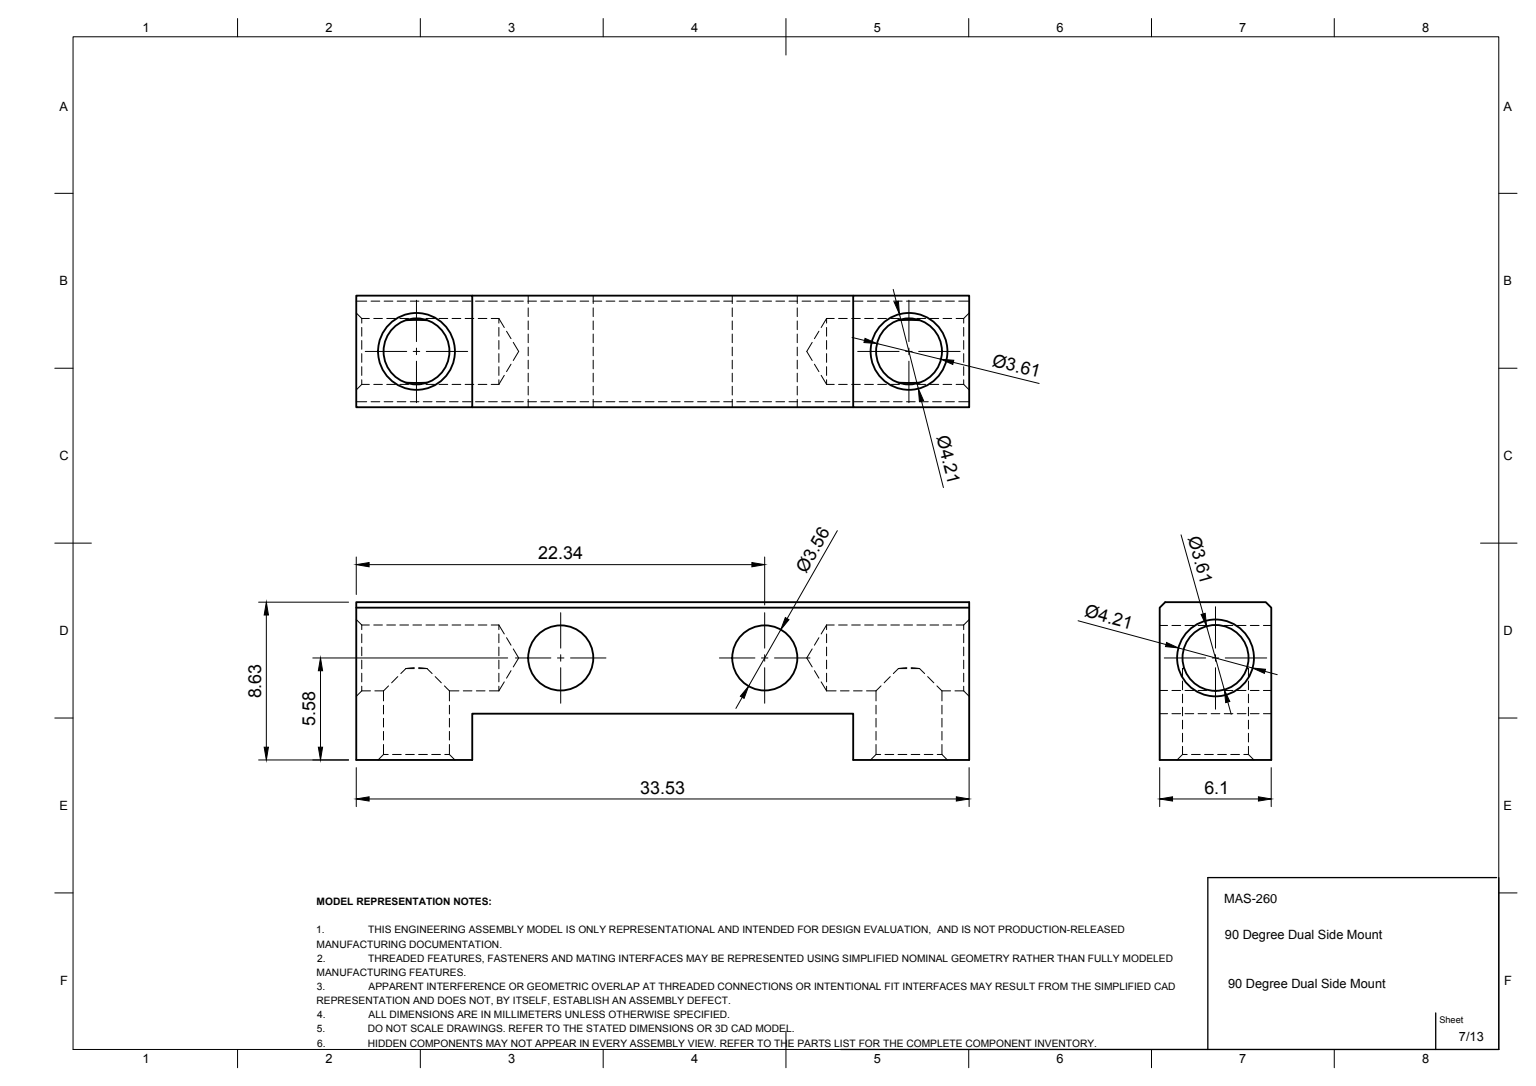
ISO-10303-21;
HEADER;
/* Generated by software containing ST-Developer
 * from STEP Tools, Inc. (www.steptools.com) 
 */

FILE_DESCRIPTION(
/* description */ (''),
/* implementation_level */ '2;1');

FILE_NAME(
/* name */ '90 Degree Dual Side Mount.step',
/* time_stamp */ '2026-10-15T13:29:10-07:00',
/* author */ (''),
/* organization */ (''),
/* preprocessor_version */ 'ST-DEVELOPER v20.2',
/* originating_system */ 'Autodesk Translation Framework v15.15.0.0',
/* authorisation */ '');

FILE_SCHEMA (('AUTOMOTIVE_DESIGN { 1 0 10303 214 3 1 1 }'));
ENDSEC;

DATA;
#10=MECHANICAL_DESIGN_GEOMETRIC_PRESENTATION_REPRESENTATION('',(#941),#83219);
#191=ELLIPSE('',#28417,2.5491199461775,1.8025);
#192=ELLIPSE('',#28419,2.5491199461775,1.8025);
#193=ELLIPSE('',#28421,2.5491199461775,1.8025);
#194=ELLIPSE('',#28427,2.5491199461775,1.8025);
#195=ELLIPSE('',#28429,2.5491199461775,1.8025);
#196=ELLIPSE('',#28431,2.5491199461775,1.8025);
#641=B_SPLINE_CURVE_WITH_KNOTS('',3,(#53054,#53055,#53056,#53057,#53058,
#53059,#53060),.UNSPECIFIED.,.F.,.F.,(4,3,4),(-0.0562125399722967,0.,0.0562125399722968),
 .UNSPECIFIED.);
#642=B_SPLINE_CURVE_WITH_KNOTS('',3,(#53062,#53063,#53064,#53065,#53066,
#53067),.UNSPECIFIED.,.F.,.F.,(4,2,4),(-0.961432950963571,-0.905220410991274,
-0.849007871018978),.UNSPECIFIED.);
#643=B_SPLINE_CURVE_WITH_KNOTS('',3,(#53077,#53078,#53079,#53080,#53081,
#53082,#53083),.UNSPECIFIED.,.F.,.F.,(4,3,4),(-0.0562125399722967,0.,0.0562125399722968),
 .UNSPECIFIED.);
#644=B_SPLINE_CURVE_WITH_KNOTS('',3,(#53085,#53086,#53087,#53088,#53089,
#53090),.UNSPECIFIED.,.F.,.F.,(4,2,4),(-0.961432950963571,-0.905220410991274,
-0.849007871018978),.UNSPECIFIED.);
#913=SHAPE_REPRESENTATION_RELATIONSHIP('SRR','None',#83308,#927);
#927=ADVANCED_BREP_SHAPE_REPRESENTATION('',(#955),#83213);
#941=STYLED_ITEM('',(#83387),#955);
#955=MANIFOLD_SOLID_BREP('Body1',#26937);
#1101=FACE_BOUND('',#4773,.T.);
#1102=FACE_BOUND('',#4777,.T.);
#1103=FACE_BOUND('',#4781,.T.);
#1104=FACE_BOUND('',#4785,.T.);
#1105=FACE_BOUND('',#4788,.T.);
#1106=FACE_BOUND('',#4792,.T.);
#1107=FACE_BOUND('',#4801,.T.);
#1108=FACE_BOUND('',#4802,.T.);
#1109=FACE_BOUND('',#4804,.T.);
#1110=FACE_BOUND('',#4805,.T.);
#1743=PLANE('',#28422);
#1744=PLANE('',#28432);
#1745=PLANE('',#28447);
#1746=PLANE('',#28451);
#1747=PLANE('',#28453);
#1748=PLANE('',#28454);
#1749=PLANE('',#28455);
#1750=PLANE('',#28456);
#1751=PLANE('',#28457);
#1752=PLANE('',#28458);
#1753=PLANE('',#28459);
#1754=PLANE('',#28460);
#2302=CYLINDRICAL_SURFACE('',#28407,1.778);
#2303=CYLINDRICAL_SURFACE('',#28410,1.778);
#2304=CYLINDRICAL_SURFACE('',#28416,1.8025);
#2305=CYLINDRICAL_SURFACE('',#28426,1.8025);
#2306=CYLINDRICAL_SURFACE('',#28435,1.8025);
#2307=CYLINDRICAL_SURFACE('',#28441,1.8025);
#3249=FACE_OUTER_BOUND('',#4768,.T.);
#3250=FACE_OUTER_BOUND('',#4769,.T.);
#3251=FACE_OUTER_BOUND('',#4770,.T.);
#3252=FACE_OUTER_BOUND('',#4771,.T.);
#3253=FACE_OUTER_BOUND('',#4772,.T.);
#3254=FACE_OUTER_BOUND('',#4774,.T.);
#3255=FACE_OUTER_BOUND('',#4775,.T.);
#3256=FACE_OUTER_BOUND('',#4776,.T.);
#3257=FACE_OUTER_BOUND('',#4778,.T.);
#3258=FACE_OUTER_BOUND('',#4779,.T.);
#3259=FACE_OUTER_BOUND('',#4780,.T.);
#3260=FACE_OUTER_BOUND('',#4782,.T.);
#3261=FACE_OUTER_BOUND('',#4783,.T.);
#3262=FACE_OUTER_BOUND('',#4784,.T.);
#3263=FACE_OUTER_BOUND('',#4786,.T.);
#3264=FACE_OUTER_BOUND('',#4787,.T.);
#3265=FACE_OUTER_BOUND('',#4789,.T.);
#3266=FACE_OUTER_BOUND('',#4790,.T.);
#3267=FACE_OUTER_BOUND('',#4791,.T.);
#3268=FACE_OUTER_BOUND('',#4793,.T.);
#3269=FACE_OUTER_BOUND('',#4794,.T.);
#3270=FACE_OUTER_BOUND('',#4795,.T.);
#3271=FACE_OUTER_BOUND('',#4796,.T.);
#3272=FACE_OUTER_BOUND('',#4797,.T.);
#3273=FACE_OUTER_BOUND('',#4798,.T.);
#3274=FACE_OUTER_BOUND('',#4799,.T.);
#3275=FACE_OUTER_BOUND('',#4800,.T.);
#3276=FACE_OUTER_BOUND('',#4803,.T.);
#4768=EDGE_LOOP('',(#22514,#22515,#22516,#22517));
#4769=EDGE_LOOP('',(#22518,#22519,#22520,#22521));
#4770=EDGE_LOOP('',(#22522,#22523,#22524,#22525));
#4771=EDGE_LOOP('',(#22526,#22527,#22528,#22529,#22530,#22531,#22532,#22533));
#4772=EDGE_LOOP('',(#22534,#22535,#22536,#22537));
#4773=EDGE_LOOP('',(#22538));
#4774=EDGE_LOOP('',(#22539,#22540,#22541,#22542));
#4775=EDGE_LOOP('',(#22543,#22544,#22545,#22546,#22547,#22548,#22549,#22550));
#4776=EDGE_LOOP('',(#22551,#22552,#22553,#22554));
#4777=EDGE_LOOP('',(#22555));
#4778=EDGE_LOOP('',(#22556,#22557));
#4779=EDGE_LOOP('',(#22558,#22559));
#4780=EDGE_LOOP('',(#22560,#22561,#22562,#22563,#22564));
#4781=EDGE_LOOP('',(#22565,#22566,#22567,#22568,#22569));
#4782=EDGE_LOOP('',(#22570,#22571));
#4783=EDGE_LOOP('',(#22572,#22573));
#4784=EDGE_LOOP('',(#22574,#22575,#22576,#22577,#22578));
#4785=EDGE_LOOP('',(#22579,#22580,#22581,#22582,#22583));
#4786=EDGE_LOOP('',(#22584,#22585,#22586,#22587));
#4787=EDGE_LOOP('',(#22588,#22589,#22590,#22591,#22592,#22593));
#4788=EDGE_LOOP('',(#22594));
#4789=EDGE_LOOP('',(#22595,#22596,#22597,#22598));
#4790=EDGE_LOOP('',(#22599,#22600,#22601,#22602));
#4791=EDGE_LOOP('',(#22603,#22604,#22605,#22606,#22607,#22608));
#4792=EDGE_LOOP('',(#22609));
#4793=EDGE_LOOP('',(#22610,#22611,#22612,#22613));
#4794=EDGE_LOOP('',(#22614,#22615,#22616,#22617));
#4795=EDGE_LOOP('',(#22618,#22619,#22620,#22621));
#4796=EDGE_LOOP('',(#22622,#22623,#22624,#22625));
#4797=EDGE_LOOP('',(#22626,#22627,#22628,#22629));
#4798=EDGE_LOOP('',(#22630,#22631,#22632,#22633));
#4799=EDGE_LOOP('',(#22634,#22635,#22636,#22637));
#4800=EDGE_LOOP('',(#22638,#22639,#22640,#22641,#22642,#22643,#22644,#22645));
#4801=EDGE_LOOP('',(#22646));
#4802=EDGE_LOOP('',(#22647));
#4803=EDGE_LOOP('',(#22648,#22649,#22650,#22651,#22652,#22653,#22654,#22655));
#4804=EDGE_LOOP('',(#22656));
#4805=EDGE_LOOP('',(#22657));
#7083=LINE('',#52991,#9594);
#7084=LINE('',#52997,#9595);
#7085=LINE('',#53003,#9596);
#7086=LINE('',#53007,#9597);
#7087=LINE('',#53020,#9598);
#7088=LINE('',#53022,#9599);
#7089=LINE('',#53024,#9600);
#7090=LINE('',#53025,#9601);
#7091=LINE('',#53030,#9602);
#7092=LINE('',#53034,#9603);
#7093=LINE('',#53047,#9604);
#7094=LINE('',#53049,#9605);
#7095=LINE('',#53051,#9606);
#7096=LINE('',#53052,#9607);
#7097=LINE('',#53072,#9608);
#7098=LINE('',#53095,#9609);
#7099=LINE('',#53101,#9610);
#7100=LINE('',#53106,#9611);
#7101=LINE('',#53108,#9612);
#7102=LINE('',#53110,#9613);
#7103=LINE('',#53111,#9614);
#7104=LINE('',#53112,#9615);
#7105=LINE('',#53115,#9616);
#7106=LINE('',#53118,#9617);
#7107=LINE('',#53123,#9618);
#7108=LINE('',#53124,#9619);
#7109=LINE('',#53126,#9620);
#7110=LINE('',#53128,#9621);
#7111=LINE('',#53129,#9622);
#7112=LINE('',#53132,#9623);
#7113=LINE('',#53134,#9624);
#7114=LINE('',#53135,#9625);
#7115=LINE('',#53137,#9626);
#7116=LINE('',#53139,#9627);
#7117=LINE('',#53142,#9628);
#7118=LINE('',#53144,#9629);
#7119=LINE('',#53145,#9630);
#7120=LINE('',#53148,#9631);
#7121=LINE('',#53150,#9632);
#7122=LINE('',#53151,#9633);
#7123=LINE('',#53153,#9634);
#7124=LINE('',#53154,#9635);
#9594=VECTOR('',#33683,1.778);
#9595=VECTOR('',#33690,1.778);
#9596=VECTOR('',#33697,1.9525);
#9597=VECTOR('',#33702,1.8025);
#9598=VECTOR('',#33715,10.);
#9599=VECTOR('',#33716,10.);
#9600=VECTOR('',#33717,10.);
#9601=VECTOR('',#33718,10.);
#9602=VECTOR('',#33723,1.9525);
#9603=VECTOR('',#33728,1.8025);
#9604=VECTOR('',#33741,10.);
#9605=VECTOR('',#33742,10.);
#9606=VECTOR('',#33743,10.);
#9607=VECTOR('',#33744,10.);
#9608=VECTOR('',#33753,1.8025);
#9609=VECTOR('',#33766,1.8025);
#9610=VECTOR('',#33773,1.9525);
#9611=VECTOR('',#33778,10.);
#9612=VECTOR('',#33779,10.);
#9613=VECTOR('',#33780,10.);
#9614=VECTOR('',#33781,10.);
#9615=VECTOR('',#33782,10.);
#9616=VECTOR('',#33785,1.8025);
#9617=VECTOR('',#33788,1.9525);
#9618=VECTOR('',#33793,10.);
#9619=VECTOR('',#33794,10.);
#9620=VECTOR('',#33795,10.);
#9621=VECTOR('',#33796,10.);
#9622=VECTOR('',#33797,10.);
#9623=VECTOR('',#33800,0.901250000000005);
#9624=VECTOR('',#33803,10.);
#9625=VECTOR('',#33804,10.);
#9626=VECTOR('',#33807,10.);
#9627=VECTOR('',#33810,10.);
#9628=VECTOR('',#33813,10.);
#9629=VECTOR('',#33814,10.);
#9630=VECTOR('',#33815,10.);
#9631=VECTOR('',#33818,10.);
#9632=VECTOR('',#33819,10.);
#9633=VECTOR('',#33820,10.);
#9634=VECTOR('',#33823,10.);
#9635=VECTOR('',#33824,10.);
#10740=CIRCLE('',#28408,1.778);
#10741=CIRCLE('',#28409,1.778);
#10742=CIRCLE('',#28411,1.778);
#10743=CIRCLE('',#28412,1.778);
#10744=CIRCLE('',#28414,1.8025);
#10745=CIRCLE('',#28415,2.1025);
#10746=CIRCLE('',#28418,1.8025);
#10747=CIRCLE('',#28420,1.8025);
#10748=CIRCLE('',#28424,1.8025);
#10749=CIRCLE('',#28425,2.1025);
#10750=CIRCLE('',#28428,1.8025);
#10751=CIRCLE('',#28430,1.8025);
#10752=CIRCLE('',#28436,1.8025);
#10753=CIRCLE('',#28437,1.8025);
#10754=CIRCLE('',#28438,1.8025);
#10755=CIRCLE('',#28442,1.8025);
#10756=CIRCLE('',#28443,1.8025);
#10757=CIRCLE('',#28444,1.8025);
#10758=CIRCLE('',#28446,2.1025);
#10759=CIRCLE('',#28450,2.1025);
#12651=VERTEX_POINT('',#52988);
#12652=VERTEX_POINT('',#52990);
#12653=VERTEX_POINT('',#52994);
#12654=VERTEX_POINT('',#52996);
#12655=VERTEX_POINT('',#53000);
#12656=VERTEX_POINT('',#53002);
#12657=VERTEX_POINT('',#53006);
#12658=VERTEX_POINT('',#53008);
#12659=VERTEX_POINT('',#53010);
#12660=VERTEX_POINT('',#53012);
#12661=VERTEX_POINT('',#53014);
#12662=VERTEX_POINT('',#53018);
#12663=VERTEX_POINT('',#53019);
#12664=VERTEX_POINT('',#53021);
#12665=VERTEX_POINT('',#53023);
#12666=VERTEX_POINT('',#53027);
#12667=VERTEX_POINT('',#53029);
#12668=VERTEX_POINT('',#53033);
#12669=VERTEX_POINT('',#53035);
#12670=VERTEX_POINT('',#53037);
#12671=VERTEX_POINT('',#53039);
#12672=VERTEX_POINT('',#53041);
#12673=VERTEX_POINT('',#53045);
#12674=VERTEX_POINT('',#53046);
#12675=VERTEX_POINT('',#53048);
#12676=VERTEX_POINT('',#53050);
#12677=VERTEX_POINT('',#53069);
#12678=VERTEX_POINT('',#53071);
#12679=VERTEX_POINT('',#53073);
#12680=VERTEX_POINT('',#53092);
#12681=VERTEX_POINT('',#53094);
#12682=VERTEX_POINT('',#53096);
#12683=VERTEX_POINT('',#53100);
#12684=VERTEX_POINT('',#53104);
#12685=VERTEX_POINT('',#53105);
#12686=VERTEX_POINT('',#53107);
#12687=VERTEX_POINT('',#53109);
#12688=VERTEX_POINT('',#53114);
#12689=VERTEX_POINT('',#53117);
#12690=VERTEX_POINT('',#53121);
#12691=VERTEX_POINT('',#53122);
#12692=VERTEX_POINT('',#53125);
#12693=VERTEX_POINT('',#53127);
#12694=VERTEX_POINT('',#53131);
#12695=VERTEX_POINT('',#53141);
#12696=VERTEX_POINT('',#53143);
#12697=VERTEX_POINT('',#53147);
#12698=VERTEX_POINT('',#53149);
#16118=EDGE_CURVE('',#12651,#12651,#10740,.T.);
#16119=EDGE_CURVE('',#12651,#12652,#7083,.T.);
#16120=EDGE_CURVE('',#12652,#12652,#10741,.T.);
#16121=EDGE_CURVE('',#12653,#12653,#10742,.T.);
#16122=EDGE_CURVE('',#12653,#12654,#7084,.T.);
#16123=EDGE_CURVE('',#12654,#12654,#10743,.T.);
#16124=EDGE_CURVE('',#12655,#12655,#10744,.T.);
#16125=EDGE_CURVE('',#12655,#12656,#7085,.T.);
#16126=EDGE_CURVE('',#12656,#12656,#10745,.T.);
#16127=EDGE_CURVE('',#12655,#12657,#7086,.T.);
#16128=EDGE_CURVE('',#12658,#12657,#191,.T.);
#16129=EDGE_CURVE('',#12658,#12659,#10746,.T.);
#16130=EDGE_CURVE('',#12660,#12659,#192,.T.);
#16131=EDGE_CURVE('',#12660,#12661,#10747,.T.);
#16132=EDGE_CURVE('',#12657,#12661,#193,.T.);
#16133=EDGE_CURVE('',#12662,#12663,#7087,.T.);
#16134=EDGE_CURVE('',#12663,#12664,#7088,.T.);
#16135=EDGE_CURVE('',#12665,#12664,#7089,.T.);
#16136=EDGE_CURVE('',#12662,#12665,#7090,.T.);
#16137=EDGE_CURVE('',#12666,#12666,#10748,.T.);
#16138=EDGE_CURVE('',#12666,#12667,#7091,.T.);
#16139=EDGE_CURVE('',#12667,#12667,#10749,.T.);
#16140=EDGE_CURVE('',#12666,#12668,#7092,.T.);
#16141=EDGE_CURVE('',#12669,#12668,#194,.T.);
#16142=EDGE_CURVE('',#12669,#12670,#10750,.T.);
#16143=EDGE_CURVE('',#12671,#12670,#195,.T.);
#16144=EDGE_CURVE('',#12671,#12672,#10751,.T.);
#16145=EDGE_CURVE('',#12668,#12672,#196,.T.);
#16146=EDGE_CURVE('',#12673,#12674,#7093,.T.);
#16147=EDGE_CURVE('',#12674,#12675,#7094,.T.);
#16148=EDGE_CURVE('',#12676,#12675,#7095,.T.);
#16149=EDGE_CURVE('',#12673,#12676,#7096,.T.);
#16150=EDGE_CURVE('',#12659,#12658,#641,.T.);
#16151=EDGE_CURVE('',#12661,#12660,#642,.T.);
#16152=EDGE_CURVE('',#12677,#12677,#10752,.T.);
#16153=EDGE_CURVE('',#12677,#12678,#7097,.T.);
#16154=EDGE_CURVE('',#12678,#12679,#10753,.T.);
#16155=EDGE_CURVE('',#12679,#12678,#10754,.T.);
#16156=EDGE_CURVE('',#12672,#12671,#643,.T.);
#16157=EDGE_CURVE('',#12670,#12669,#644,.T.);
#16158=EDGE_CURVE('',#12680,#12680,#10755,.T.);
#16159=EDGE_CURVE('',#12680,#12681,#7098,.T.);
#16160=EDGE_CURVE('',#12681,#12682,#10756,.T.);
#16161=EDGE_CURVE('',#12682,#12681,#10757,.T.);
#16162=EDGE_CURVE('',#12677,#12683,#7099,.T.);
#16163=EDGE_CURVE('',#12683,#12683,#10758,.T.);
#16164=EDGE_CURVE('',#12684,#12685,#7100,.T.);
#16165=EDGE_CURVE('',#12686,#12684,#7101,.T.);
#16166=EDGE_CURVE('',#12687,#12686,#7102,.T.);
#16167=EDGE_CURVE('',#12687,#12662,#7103,.T.);
#16168=EDGE_CURVE('',#12685,#12665,#7104,.T.);
#16169=EDGE_CURVE('',#12688,#12679,#7105,.T.);
#16170=EDGE_CURVE('',#12680,#12689,#7106,.T.);
#16171=EDGE_CURVE('',#12689,#12689,#10759,.T.);
#16172=EDGE_CURVE('',#12690,#12691,#7107,.T.);
#16173=EDGE_CURVE('',#12675,#12690,#7108,.T.);
#16174=EDGE_CURVE('',#12674,#12692,#7109,.T.);
#16175=EDGE_CURVE('',#12693,#12692,#7110,.T.);
#16176=EDGE_CURVE('',#12693,#12691,#7111,.T.);
#16177=EDGE_CURVE('',#12694,#12682,#7112,.T.);
#16178=EDGE_CURVE('',#12685,#12690,#7113,.T.);
#16179=EDGE_CURVE('',#12691,#12684,#7114,.T.);
#16180=EDGE_CURVE('',#12686,#12693,#7115,.T.);
#16181=EDGE_CURVE('',#12692,#12687,#7116,.T.);
#16182=EDGE_CURVE('',#12695,#12673,#7117,.T.);
#16183=EDGE_CURVE('',#12696,#12676,#7118,.T.);
#16184=EDGE_CURVE('',#12695,#12696,#7119,.T.);
#16185=EDGE_CURVE('',#12697,#12695,#7120,.T.);
#16186=EDGE_CURVE('',#12698,#12696,#7121,.T.);
#16187=EDGE_CURVE('',#12697,#12698,#7122,.T.);
#16188=EDGE_CURVE('',#12663,#12697,#7123,.T.);
#16189=EDGE_CURVE('',#12664,#12698,#7124,.T.);
#22514=ORIENTED_EDGE('',*,*,#16118,.F.);
#22515=ORIENTED_EDGE('',*,*,#16119,.T.);
#22516=ORIENTED_EDGE('',*,*,#16120,.F.);
#22517=ORIENTED_EDGE('',*,*,#16119,.F.);
#22518=ORIENTED_EDGE('',*,*,#16121,.F.);
#22519=ORIENTED_EDGE('',*,*,#16122,.T.);
#22520=ORIENTED_EDGE('',*,*,#16123,.F.);
#22521=ORIENTED_EDGE('',*,*,#16122,.F.);
#22522=ORIENTED_EDGE('',*,*,#16124,.T.);
#22523=ORIENTED_EDGE('',*,*,#16125,.T.);
#22524=ORIENTED_EDGE('',*,*,#16126,.T.);
#22525=ORIENTED_EDGE('',*,*,#16125,.F.);
#22526=ORIENTED_EDGE('',*,*,#16124,.F.);
#22527=ORIENTED_EDGE('',*,*,#16127,.T.);
#22528=ORIENTED_EDGE('',*,*,#16128,.F.);
#22529=ORIENTED_EDGE('',*,*,#16129,.T.);
#22530=ORIENTED_EDGE('',*,*,#16130,.F.);
#22531=ORIENTED_EDGE('',*,*,#16131,.T.);
#22532=ORIENTED_EDGE('',*,*,#16132,.F.);
#22533=ORIENTED_EDGE('',*,*,#16127,.F.);
#22534=ORIENTED_EDGE('',*,*,#16133,.T.);
#22535=ORIENTED_EDGE('',*,*,#16134,.T.);
#22536=ORIENTED_EDGE('',*,*,#16135,.F.);
#22537=ORIENTED_EDGE('',*,*,#16136,.F.);
#22538=ORIENTED_EDGE('',*,*,#16126,.F.);
#22539=ORIENTED_EDGE('',*,*,#16137,.T.);
#22540=ORIENTED_EDGE('',*,*,#16138,.T.);
#22541=ORIENTED_EDGE('',*,*,#16139,.T.);
#22542=ORIENTED_EDGE('',*,*,#16138,.F.);
#22543=ORIENTED_EDGE('',*,*,#16137,.F.);
#22544=ORIENTED_EDGE('',*,*,#16140,.T.);
#22545=ORIENTED_EDGE('',*,*,#16141,.F.);
#22546=ORIENTED_EDGE('',*,*,#16142,.T.);
#22547=ORIENTED_EDGE('',*,*,#16143,.F.);
#22548=ORIENTED_EDGE('',*,*,#16144,.T.);
#22549=ORIENTED_EDGE('',*,*,#16145,.F.);
#22550=ORIENTED_EDGE('',*,*,#16140,.F.);
#22551=ORIENTED_EDGE('',*,*,#16146,.T.);
#22552=ORIENTED_EDGE('',*,*,#16147,.T.);
#22553=ORIENTED_EDGE('',*,*,#16148,.F.);
#22554=ORIENTED_EDGE('',*,*,#16149,.F.);
#22555=ORIENTED_EDGE('',*,*,#16139,.F.);
#22556=ORIENTED_EDGE('',*,*,#16150,.F.);
#22557=ORIENTED_EDGE('',*,*,#16129,.F.);
#22558=ORIENTED_EDGE('',*,*,#16151,.F.);
#22559=ORIENTED_EDGE('',*,*,#16131,.F.);
#22560=ORIENTED_EDGE('',*,*,#16152,.F.);
#22561=ORIENTED_EDGE('',*,*,#16153,.T.);
#22562=ORIENTED_EDGE('',*,*,#16154,.T.);
#22563=ORIENTED_EDGE('',*,*,#16155,.T.);
#22564=ORIENTED_EDGE('',*,*,#16153,.F.);
#22565=ORIENTED_EDGE('',*,*,#16151,.T.);
#22566=ORIENTED_EDGE('',*,*,#16130,.T.);
#22567=ORIENTED_EDGE('',*,*,#16150,.T.);
#22568=ORIENTED_EDGE('',*,*,#16128,.T.);
#22569=ORIENTED_EDGE('',*,*,#16132,.T.);
#22570=ORIENTED_EDGE('',*,*,#16156,.F.);
#22571=ORIENTED_EDGE('',*,*,#16144,.F.);
#22572=ORIENTED_EDGE('',*,*,#16157,.F.);
#22573=ORIENTED_EDGE('',*,*,#16142,.F.);
#22574=ORIENTED_EDGE('',*,*,#16158,.F.);
#22575=ORIENTED_EDGE('',*,*,#16159,.T.);
#22576=ORIENTED_EDGE('',*,*,#16160,.T.);
#22577=ORIENTED_EDGE('',*,*,#16161,.T.);
#22578=ORIENTED_EDGE('',*,*,#16159,.F.);
#22579=ORIENTED_EDGE('',*,*,#16157,.T.);
#22580=ORIENTED_EDGE('',*,*,#16141,.T.);
#22581=ORIENTED_EDGE('',*,*,#16145,.T.);
#22582=ORIENTED_EDGE('',*,*,#16156,.T.);
#22583=ORIENTED_EDGE('',*,*,#16143,.T.);
#22584=ORIENTED_EDGE('',*,*,#16152,.T.);
#22585=ORIENTED_EDGE('',*,*,#16162,.T.);
#22586=ORIENTED_EDGE('',*,*,#16163,.T.);
#22587=ORIENTED_EDGE('',*,*,#16162,.F.);
#22588=ORIENTED_EDGE('',*,*,#16164,.F.);
#22589=ORIENTED_EDGE('',*,*,#16165,.F.);
#22590=ORIENTED_EDGE('',*,*,#16166,.F.);
#22591=ORIENTED_EDGE('',*,*,#16167,.T.);
#22592=ORIENTED_EDGE('',*,*,#16136,.T.);
#22593=ORIENTED_EDGE('',*,*,#16168,.F.);
#22594=ORIENTED_EDGE('',*,*,#16163,.F.);
#22595=ORIENTED_EDGE('',*,*,#16169,.T.);
#22596=ORIENTED_EDGE('',*,*,#16154,.F.);
#22597=ORIENTED_EDGE('',*,*,#16155,.F.);
#22598=ORIENTED_EDGE('',*,*,#16169,.F.);
#22599=ORIENTED_EDGE('',*,*,#16158,.T.);
#22600=ORIENTED_EDGE('',*,*,#16170,.T.);
#22601=ORIENTED_EDGE('',*,*,#16171,.T.);
#22602=ORIENTED_EDGE('',*,*,#16170,.F.);
#22603=ORIENTED_EDGE('',*,*,#16172,.F.);
#22604=ORIENTED_EDGE('',*,*,#16173,.F.);
#22605=ORIENTED_EDGE('',*,*,#16147,.F.);
#22606=ORIENTED_EDGE('',*,*,#16174,.T.);
#22607=ORIENTED_EDGE('',*,*,#16175,.F.);
#22608=ORIENTED_EDGE('',*,*,#16176,.T.);
#22609=ORIENTED_EDGE('',*,*,#16171,.F.);
#22610=ORIENTED_EDGE('',*,*,#16177,.T.);
#22611=ORIENTED_EDGE('',*,*,#16160,.F.);
#22612=ORIENTED_EDGE('',*,*,#16161,.F.);
#22613=ORIENTED_EDGE('',*,*,#16177,.F.);
#22614=ORIENTED_EDGE('',*,*,#16164,.T.);
#22615=ORIENTED_EDGE('',*,*,#16178,.T.);
#22616=ORIENTED_EDGE('',*,*,#16172,.T.);
#22617=ORIENTED_EDGE('',*,*,#16179,.T.);
#22618=ORIENTED_EDGE('',*,*,#16179,.F.);
#22619=ORIENTED_EDGE('',*,*,#16176,.F.);
#22620=ORIENTED_EDGE('',*,*,#16180,.F.);
#22621=ORIENTED_EDGE('',*,*,#16165,.T.);
#22622=ORIENTED_EDGE('',*,*,#16166,.T.);
#22623=ORIENTED_EDGE('',*,*,#16180,.T.);
#22624=ORIENTED_EDGE('',*,*,#16175,.T.);
#22625=ORIENTED_EDGE('',*,*,#16181,.T.);
#22626=ORIENTED_EDGE('',*,*,#16182,.T.);
#22627=ORIENTED_EDGE('',*,*,#16149,.T.);
#22628=ORIENTED_EDGE('',*,*,#16183,.F.);
#22629=ORIENTED_EDGE('',*,*,#16184,.F.);
#22630=ORIENTED_EDGE('',*,*,#16185,.T.);
#22631=ORIENTED_EDGE('',*,*,#16184,.T.);
#22632=ORIENTED_EDGE('',*,*,#16186,.F.);
#22633=ORIENTED_EDGE('',*,*,#16187,.F.);
#22634=ORIENTED_EDGE('',*,*,#16188,.T.);
#22635=ORIENTED_EDGE('',*,*,#16187,.T.);
#22636=ORIENTED_EDGE('',*,*,#16189,.F.);
#22637=ORIENTED_EDGE('',*,*,#16134,.F.);
#22638=ORIENTED_EDGE('',*,*,#16178,.F.);
#22639=ORIENTED_EDGE('',*,*,#16168,.T.);
#22640=ORIENTED_EDGE('',*,*,#16135,.T.);
#22641=ORIENTED_EDGE('',*,*,#16189,.T.);
#22642=ORIENTED_EDGE('',*,*,#16186,.T.);
#22643=ORIENTED_EDGE('',*,*,#16183,.T.);
#22644=ORIENTED_EDGE('',*,*,#16148,.T.);
#22645=ORIENTED_EDGE('',*,*,#16173,.T.);
#22646=ORIENTED_EDGE('',*,*,#16120,.T.);
#22647=ORIENTED_EDGE('',*,*,#16123,.T.);
#22648=ORIENTED_EDGE('',*,*,#16181,.F.);
#22649=ORIENTED_EDGE('',*,*,#16174,.F.);
#22650=ORIENTED_EDGE('',*,*,#16146,.F.);
#22651=ORIENTED_EDGE('',*,*,#16182,.F.);
#22652=ORIENTED_EDGE('',*,*,#16185,.F.);
#22653=ORIENTED_EDGE('',*,*,#16188,.F.);
#22654=ORIENTED_EDGE('',*,*,#16133,.F.);
#22655=ORIENTED_EDGE('',*,*,#16167,.F.);
#22656=ORIENTED_EDGE('',*,*,#16118,.T.);
#22657=ORIENTED_EDGE('',*,*,#16121,.T.);
#25526=CONICAL_SURFACE('',#28413,1.9525,0.785398163397452);
#25527=CONICAL_SURFACE('',#28423,1.9525,0.785398163397452);
#25528=CONICAL_SURFACE('',#28433,0.90125,1.02974425867665);
#25529=CONICAL_SURFACE('',#28434,0.90125,1.02974425867665);
#25530=CONICAL_SURFACE('',#28439,0.90125,1.02974425867665);
#25531=CONICAL_SURFACE('',#28440,0.90125,1.02974425867665);
#25532=CONICAL_SURFACE('',#28445,1.9525,0.785398163397448);
#25533=CONICAL_SURFACE('',#28448,1.8025,1.02974425867665);
#25534=CONICAL_SURFACE('',#28449,1.9525,0.785398163397448);
#25535=CONICAL_SURFACE('',#28452,0.901250000000005,1.02974425867665);
#26442=ADVANCED_FACE('',(#3249),#2302,.F.);
#26443=ADVANCED_FACE('',(#3250),#2303,.F.);
#26444=ADVANCED_FACE('',(#3251),#25526,.F.);
#26445=ADVANCED_FACE('',(#3252),#2304,.F.);
#26446=ADVANCED_FACE('',(#3253,#1101),#1743,.T.);
#26447=ADVANCED_FACE('',(#3254),#25527,.F.);
#26448=ADVANCED_FACE('',(#3255),#2305,.F.);
#26449=ADVANCED_FACE('',(#3256,#1102),#1744,.T.);
#26450=ADVANCED_FACE('',(#3257),#25528,.F.);
#26451=ADVANCED_FACE('',(#3258),#25529,.F.);
#26452=ADVANCED_FACE('',(#3259,#1103),#2306,.F.);
#26453=ADVANCED_FACE('',(#3260),#25530,.F.);
#26454=ADVANCED_FACE('',(#3261),#25531,.F.);
#26455=ADVANCED_FACE('',(#3262,#1104),#2307,.F.);
#26456=ADVANCED_FACE('',(#3263),#25532,.F.);
#26457=ADVANCED_FACE('',(#3264,#1105),#1745,.T.);
#26458=ADVANCED_FACE('',(#3265),#25533,.F.);
#26459=ADVANCED_FACE('',(#3266),#25534,.F.);
#26460=ADVANCED_FACE('',(#3267,#1106),#1746,.T.);
#26461=ADVANCED_FACE('',(#3268),#25535,.F.);
#26462=ADVANCED_FACE('',(#3269),#1747,.T.);
#26463=ADVANCED_FACE('',(#3270),#1748,.T.);
#26464=ADVANCED_FACE('',(#3271),#1749,.T.);
#26465=ADVANCED_FACE('',(#3272),#1750,.T.);
#26466=ADVANCED_FACE('',(#3273),#1751,.T.);
#26467=ADVANCED_FACE('',(#3274),#1752,.T.);
#26468=ADVANCED_FACE('',(#3275,#1107,#1108),#1753,.T.);
#26469=ADVANCED_FACE('',(#3276,#1109,#1110),#1754,.F.);
#26937=CLOSED_SHELL('',(#26442,#26443,#26444,#26445,#26446,#26447,#26448,
#26449,#26450,#26451,#26452,#26453,#26454,#26455,#26456,#26457,#26458,#26459,
#26460,#26461,#26462,#26463,#26464,#26465,#26466,#26467,#26468,#26469));
#28406=AXIS2_PLACEMENT_3D('',#52986,#33677,#33678);
#28407=AXIS2_PLACEMENT_3D('',#52987,#33679,#33680);
#28408=AXIS2_PLACEMENT_3D('',#52989,#33681,#33682);
#28409=AXIS2_PLACEMENT_3D('',#52992,#33684,#33685);
#28410=AXIS2_PLACEMENT_3D('',#52993,#33686,#33687);
#28411=AXIS2_PLACEMENT_3D('',#52995,#33688,#33689);
#28412=AXIS2_PLACEMENT_3D('',#52998,#33691,#33692);
#28413=AXIS2_PLACEMENT_3D('',#52999,#33693,#33694);
#28414=AXIS2_PLACEMENT_3D('',#53001,#33695,#33696);
#28415=AXIS2_PLACEMENT_3D('',#53004,#33698,#33699);
#28416=AXIS2_PLACEMENT_3D('',#53005,#33700,#33701);
#28417=AXIS2_PLACEMENT_3D('',#53009,#33703,#33704);
#28418=AXIS2_PLACEMENT_3D('',#53011,#33705,#33706);
#28419=AXIS2_PLACEMENT_3D('',#53013,#33707,#33708);
#28420=AXIS2_PLACEMENT_3D('',#53015,#33709,#33710);
#28421=AXIS2_PLACEMENT_3D('',#53016,#33711,#33712);
#28422=AXIS2_PLACEMENT_3D('',#53017,#33713,#33714);
#28423=AXIS2_PLACEMENT_3D('',#53026,#33719,#33720);
#28424=AXIS2_PLACEMENT_3D('',#53028,#33721,#33722);
#28425=AXIS2_PLACEMENT_3D('',#53031,#33724,#33725);
#28426=AXIS2_PLACEMENT_3D('',#53032,#33726,#33727);
#28427=AXIS2_PLACEMENT_3D('',#53036,#33729,#33730);
#28428=AXIS2_PLACEMENT_3D('',#53038,#33731,#33732);
#28429=AXIS2_PLACEMENT_3D('',#53040,#33733,#33734);
#28430=AXIS2_PLACEMENT_3D('',#53042,#33735,#33736);
#28431=AXIS2_PLACEMENT_3D('',#53043,#33737,#33738);
#28432=AXIS2_PLACEMENT_3D('',#53044,#33739,#33740);
#28433=AXIS2_PLACEMENT_3D('',#53053,#33745,#33746);
#28434=AXIS2_PLACEMENT_3D('',#53061,#33747,#33748);
#28435=AXIS2_PLACEMENT_3D('',#53068,#33749,#33750);
#28436=AXIS2_PLACEMENT_3D('',#53070,#33751,#33752);
#28437=AXIS2_PLACEMENT_3D('',#53074,#33754,#33755);
#28438=AXIS2_PLACEMENT_3D('',#53075,#33756,#33757);
#28439=AXIS2_PLACEMENT_3D('',#53076,#33758,#33759);
#28440=AXIS2_PLACEMENT_3D('',#53084,#33760,#33761);
#28441=AXIS2_PLACEMENT_3D('',#53091,#33762,#33763);
#28442=AXIS2_PLACEMENT_3D('',#53093,#33764,#33765);
#28443=AXIS2_PLACEMENT_3D('',#53097,#33767,#33768);
#28444=AXIS2_PLACEMENT_3D('',#53098,#33769,#33770);
#28445=AXIS2_PLACEMENT_3D('',#53099,#33771,#33772);
#28446=AXIS2_PLACEMENT_3D('',#53102,#33774,#33775);
#28447=AXIS2_PLACEMENT_3D('',#53103,#33776,#33777);
#28448=AXIS2_PLACEMENT_3D('',#53113,#33783,#33784);
#28449=AXIS2_PLACEMENT_3D('',#53116,#33786,#33787);
#28450=AXIS2_PLACEMENT_3D('',#53119,#33789,#33790);
#28451=AXIS2_PLACEMENT_3D('',#53120,#33791,#33792);
#28452=AXIS2_PLACEMENT_3D('',#53130,#33798,#33799);
#28453=AXIS2_PLACEMENT_3D('',#53133,#33801,#33802);
#28454=AXIS2_PLACEMENT_3D('',#53136,#33805,#33806);
#28455=AXIS2_PLACEMENT_3D('',#53138,#33808,#33809);
#28456=AXIS2_PLACEMENT_3D('',#53140,#33811,#33812);
#28457=AXIS2_PLACEMENT_3D('',#53146,#33816,#33817);
#28458=AXIS2_PLACEMENT_3D('',#53152,#33821,#33822);
#28459=AXIS2_PLACEMENT_3D('',#53155,#33825,#33826);
#28460=AXIS2_PLACEMENT_3D('',#53156,#33827,#33828);
#33677=DIRECTION('axis',(0.,0.,1.));
#33678=DIRECTION('refdir',(1.,0.,0.));
#33679=DIRECTION('center_axis',(0.,0.,1.));
#33680=DIRECTION('ref_axis',(1.,0.,0.));
#33681=DIRECTION('center_axis',(0.,0.,1.));
#33682=DIRECTION('ref_axis',(1.,0.,0.));
#33683=DIRECTION('',(0.,0.,1.));
#33684=DIRECTION('center_axis',(0.,0.,-1.));
#33685=DIRECTION('ref_axis',(1.,0.,0.));
#33686=DIRECTION('center_axis',(0.,0.,1.));
#33687=DIRECTION('ref_axis',(1.,0.,0.));
#33688=DIRECTION('center_axis',(0.,0.,1.));
#33689=DIRECTION('ref_axis',(1.,0.,0.));
#33690=DIRECTION('',(0.,0.,1.));
#33691=DIRECTION('center_axis',(0.,0.,-1.));
#33692=DIRECTION('ref_axis',(1.,0.,0.));
#33693=DIRECTION('center_axis',(0.,-1.,0.));
#33694=DIRECTION('ref_axis',(1.,0.,0.));
#33695=DIRECTION('center_axis',(0.,1.,0.));
#33696=DIRECTION('ref_axis',(1.,0.,0.));
#33697=DIRECTION('',(-0.70710678118655,-0.707106781186545,-8.65956056235497E-17));
#33698=DIRECTION('center_axis',(0.,-1.,0.));
#33699=DIRECTION('ref_axis',(1.,0.,0.));
#33700=DIRECTION('center_axis',(0.,1.,0.));
#33701=DIRECTION('ref_axis',(1.,0.,0.));
#33702=DIRECTION('',(0.,1.,0.));
#33703=DIRECTION('center_axis',(0.707106781186548,-0.707106781186548,0.));
#33704=DIRECTION('ref_axis',(0.707106781186548,0.707106781186548,0.));
#33705=DIRECTION('center_axis',(0.,1.,0.));
#33706=DIRECTION('ref_axis',(1.,0.,0.));
#33707=DIRECTION('center_axis',(-0.707106781186548,-0.707106781186548,0.));
#33708=DIRECTION('ref_axis',(0.707106781186548,-0.707106781186548,0.));
#33709=DIRECTION('center_axis',(0.,1.,0.));
#33710=DIRECTION('ref_axis',(1.,0.,0.));
#33711=DIRECTION('center_axis',(0.707106781186548,-0.707106781186548,0.));
#33712=DIRECTION('ref_axis',(0.707106781186548,0.707106781186548,0.));
#33713=DIRECTION('center_axis',(0.,-1.,0.));
#33714=DIRECTION('ref_axis',(1.,0.,0.));
#33715=DIRECTION('',(1.,0.,0.));
#33716=DIRECTION('',(0.,0.,1.));
#33717=DIRECTION('',(1.,0.,0.));
#33718=DIRECTION('',(0.,0.,1.));
#33719=DIRECTION('center_axis',(0.,-1.,0.));
#33720=DIRECTION('ref_axis',(1.,0.,0.));
#33721=DIRECTION('center_axis',(0.,1.,0.));
#33722=DIRECTION('ref_axis',(1.,0.,0.));
#33723=DIRECTION('',(-0.70710678118655,-0.707106781186545,-8.65956056235497E-17));
#33724=DIRECTION('center_axis',(0.,-1.,0.));
#33725=DIRECTION('ref_axis',(1.,0.,0.));
#33726=DIRECTION('center_axis',(0.,1.,0.));
#33727=DIRECTION('ref_axis',(1.,0.,0.));
#33728=DIRECTION('',(0.,1.,0.));
#33729=DIRECTION('center_axis',(0.707106781186548,-0.707106781186548,0.));
#33730=DIRECTION('ref_axis',(0.707106781186548,0.707106781186548,0.));
#33731=DIRECTION('center_axis',(0.,1.,0.));
#33732=DIRECTION('ref_axis',(1.,0.,0.));
#33733=DIRECTION('center_axis',(-0.707106781186548,-0.707106781186548,0.));
#33734=DIRECTION('ref_axis',(0.707106781186548,-0.707106781186548,0.));
#33735=DIRECTION('center_axis',(0.,1.,0.));
#33736=DIRECTION('ref_axis',(1.,0.,0.));
#33737=DIRECTION('center_axis',(0.707106781186548,-0.707106781186548,0.));
#33738=DIRECTION('ref_axis',(0.707106781186548,0.707106781186548,0.));
#33739=DIRECTION('center_axis',(0.,-1.,0.));
#33740=DIRECTION('ref_axis',(1.,0.,0.));
#33741=DIRECTION('',(1.,0.,0.));
#33742=DIRECTION('',(0.,0.,1.));
#33743=DIRECTION('',(1.,0.,0.));
#33744=DIRECTION('',(0.,0.,1.));
#33745=DIRECTION('center_axis',(0.,-1.,0.));
#33746=DIRECTION('ref_axis',(1.,0.,0.));
#33747=DIRECTION('center_axis',(0.,-1.,0.));
#33748=DIRECTION('ref_axis',(1.,0.,0.));
#33749=DIRECTION('center_axis',(1.,0.,0.));
#33750=DIRECTION('ref_axis',(0.,0.,-1.));
#33751=DIRECTION('center_axis',(1.,0.,0.));
#33752=DIRECTION('ref_axis',(0.,0.,-1.));
#33753=DIRECTION('',(1.,0.,0.));
#33754=DIRECTION('center_axis',(1.,0.,0.));
#33755=DIRECTION('ref_axis',(0.,0.,-1.));
#33756=DIRECTION('center_axis',(1.,0.,0.));
#33757=DIRECTION('ref_axis',(0.,0.,-1.));
#33758=DIRECTION('center_axis',(0.,-1.,0.));
#33759=DIRECTION('ref_axis',(1.,0.,0.));
#33760=DIRECTION('center_axis',(0.,-1.,0.));
#33761=DIRECTION('ref_axis',(1.,0.,0.));
#33762=DIRECTION('center_axis',(-1.,0.,0.));
#33763=DIRECTION('ref_axis',(0.,0.,-1.));
#33764=DIRECTION('center_axis',(-1.,0.,0.));
#33765=DIRECTION('ref_axis',(0.,0.,-1.));
#33766=DIRECTION('',(-1.,0.,0.));
#33767=DIRECTION('center_axis',(-1.,0.,0.));
#33768=DIRECTION('ref_axis',(0.,0.,-1.));
#33769=DIRECTION('center_axis',(-1.,0.,0.));
#33770=DIRECTION('ref_axis',(0.,0.,-1.));
#33771=DIRECTION('center_axis',(-1.,0.,0.));
#33772=DIRECTION('ref_axis',(0.,0.,-1.));
#33773=DIRECTION('',(-0.707106781186548,8.65956056235493E-17,0.707106781186547));
#33774=DIRECTION('center_axis',(-1.,0.,0.));
#33775=DIRECTION('ref_axis',(0.,0.,-1.));
#33776=DIRECTION('center_axis',(-1.,0.,0.));
#33777=DIRECTION('ref_axis',(0.,-1.,0.));
#33778=DIRECTION('',(0.,-0.707106781186553,0.707106781186542));
#33779=DIRECTION('',(0.,0.,1.));
#33780=DIRECTION('',(0.,0.70710678118655,0.707106781186545));
#33781=DIRECTION('',(0.,-1.,0.));
#33782=DIRECTION('',(0.,-1.,0.));
#33783=DIRECTION('center_axis',(-1.,0.,0.));
#33784=DIRECTION('ref_axis',(0.,1.,0.));
#33785=DIRECTION('',(-0.515038074910058,-0.85716730070211,1.04972719113862E-16));
#33786=DIRECTION('center_axis',(1.,0.,0.));
#33787=DIRECTION('ref_axis',(0.,0.,-1.));
#33788=DIRECTION('',(0.707106781186548,-8.65956056235493E-17,0.707106781186547));
#33789=DIRECTION('center_axis',(1.,0.,0.));
#33790=DIRECTION('ref_axis',(0.,0.,-1.));
#33791=DIRECTION('center_axis',(1.,0.,0.));
#33792=DIRECTION('ref_axis',(0.,1.,0.));
#33793=DIRECTION('',(0.,0.707106781186553,-0.707106781186542));
#33794=DIRECTION('',(0.,1.,0.));
#33795=DIRECTION('',(0.,1.,0.));
#33796=DIRECTION('',(0.,-0.70710678118655,-0.707106781186545));
#33797=DIRECTION('',(0.,0.,1.));
#33798=DIRECTION('center_axis',(1.,0.,0.));
#33799=DIRECTION('ref_axis',(0.,1.,0.));
#33800=DIRECTION('',(0.515038074910058,-0.85716730070211,-1.04972719113862E-16));
#33801=DIRECTION('center_axis',(0.,0.707106781186542,0.707106781186553));
#33802=DIRECTION('ref_axis',(1.,0.,0.));
#33803=DIRECTION('',(1.,0.,0.));
#33804=DIRECTION('',(-1.,0.,0.));
#33805=DIRECTION('center_axis',(0.,1.,0.));
#33806=DIRECTION('ref_axis',(-1.,0.,0.));
#33807=DIRECTION('',(1.,0.,0.));
#33808=DIRECTION('center_axis',(0.,0.707106781186545,-0.70710678118655));
#33809=DIRECTION('ref_axis',(-1.,0.,0.));
#33810=DIRECTION('',(-1.,0.,0.));
#33811=DIRECTION('center_axis',(-1.,0.,0.));
#33812=DIRECTION('ref_axis',(0.,-1.,0.));
#33813=DIRECTION('',(0.,-1.,0.));
#33814=DIRECTION('',(0.,-1.,0.));
#33815=DIRECTION('',(0.,0.,1.));
#33816=DIRECTION('center_axis',(0.,-1.,0.));
#33817=DIRECTION('ref_axis',(1.,0.,0.));
#33818=DIRECTION('',(1.,0.,0.));
#33819=DIRECTION('',(1.,0.,0.));
#33820=DIRECTION('',(0.,0.,1.));
#33821=DIRECTION('center_axis',(1.,0.,0.));
#33822=DIRECTION('ref_axis',(0.,1.,0.));
#33823=DIRECTION('',(0.,1.,0.));
#33824=DIRECTION('',(0.,1.,0.));
#33825=DIRECTION('center_axis',(0.,0.,1.));
#33826=DIRECTION('ref_axis',(1.,0.,0.));
#33827=DIRECTION('center_axis',(0.,0.,1.));
#33828=DIRECTION('ref_axis',(1.,0.,0.));
#52986=CARTESIAN_POINT('',(0.,0.,0.));
#52987=CARTESIAN_POINT('Origin',(5.58,44.696,15.24));
#52988=CARTESIAN_POINT('',(3.802,44.696,15.24));
#52989=CARTESIAN_POINT('Origin',(5.58,44.696,15.24));
#52990=CARTESIAN_POINT('',(3.802,44.696,21.34));
#52991=CARTESIAN_POINT('',(3.802,44.696,15.24));
#52992=CARTESIAN_POINT('Origin',(5.58,44.696,21.34));
#52993=CARTESIAN_POINT('Origin',(-5.58,44.696,15.24));
#52994=CARTESIAN_POINT('',(-7.358,44.696,15.24));
#52995=CARTESIAN_POINT('Origin',(-5.58,44.696,15.24));
#52996=CARTESIAN_POINT('',(-7.358,44.696,21.34));
#52997=CARTESIAN_POINT('',(-7.358,44.696,15.24));
#52998=CARTESIAN_POINT('Origin',(-5.58,44.696,21.34));
#52999=CARTESIAN_POINT('Origin',(-13.47,39.266,18.29));
#53000=CARTESIAN_POINT('',(-15.2725,39.416,18.29));
#53001=CARTESIAN_POINT('Origin',(-13.47,39.416,18.29));
#53002=CARTESIAN_POINT('',(-15.5725,39.116,18.29));
#53003=CARTESIAN_POINT('',(-15.4225,39.266,18.29));
#53004=CARTESIAN_POINT('Origin',(-13.47,39.116,18.29));
#53005=CARTESIAN_POINT('Origin',(-13.47,39.116,18.29));
#53006=CARTESIAN_POINT('',(-15.2725,42.8935,18.29));
#53007=CARTESIAN_POINT('',(-15.2725,39.116,18.29));
#53008=CARTESIAN_POINT('',(-14.05,44.116,19.9966359453615));
#53009=CARTESIAN_POINT('Origin',(-13.47,44.696,18.29));
#53010=CARTESIAN_POINT('',(-12.89,44.116,19.9966359453615));
#53011=CARTESIAN_POINT('Origin',(-13.47,44.116,18.29));
#53012=CARTESIAN_POINT('',(-12.89,44.116,16.5833640546385));
#53013=CARTESIAN_POINT('Origin',(-13.47,44.696,18.29));
#53014=CARTESIAN_POINT('',(-14.05,44.116,16.5833640546385));
#53015=CARTESIAN_POINT('Origin',(-13.47,44.116,18.29));
#53016=CARTESIAN_POINT('Origin',(-13.47,44.696,18.29));
#53017=CARTESIAN_POINT('Origin',(-16.764,39.116,15.24));
#53018=CARTESIAN_POINT('',(-16.764,39.116,15.24));
#53019=CARTESIAN_POINT('',(-10.42,39.116,15.24));
#53020=CARTESIAN_POINT('',(-16.764,39.116,15.24));
#53021=CARTESIAN_POINT('',(-10.42,39.116,21.34));
#53022=CARTESIAN_POINT('',(-10.42,39.116,15.24));
#53023=CARTESIAN_POINT('',(-16.764,39.116,21.34));
#53024=CARTESIAN_POINT('',(-16.764,39.116,21.34));
#53025=CARTESIAN_POINT('',(-16.764,39.116,15.24));
#53026=CARTESIAN_POINT('Origin',(13.47,39.266,18.29));
#53027=CARTESIAN_POINT('',(11.6675,39.416,18.29));
#53028=CARTESIAN_POINT('Origin',(13.47,39.416,18.29));
#53029=CARTESIAN_POINT('',(11.3675,39.116,18.29));
#53030=CARTESIAN_POINT('',(11.5175,39.266,18.29));
#53031=CARTESIAN_POINT('Origin',(13.47,39.116,18.29));
#53032=CARTESIAN_POINT('Origin',(13.47,39.116,18.29));
#53033=CARTESIAN_POINT('',(11.6675,42.8935,18.29));
#53034=CARTESIAN_POINT('',(11.6675,39.116,18.29));
#53035=CARTESIAN_POINT('',(12.89,44.116,19.9966359453615));
#53036=CARTESIAN_POINT('Origin',(13.47,44.696,18.29));
#53037=CARTESIAN_POINT('',(14.05,44.116,19.9966359453615));
#53038=CARTESIAN_POINT('Origin',(13.47,44.116,18.29));
#53039=CARTESIAN_POINT('',(14.05,44.116,16.5833640546385));
#53040=CARTESIAN_POINT('Origin',(13.47,44.696,18.29));
#53041=CARTESIAN_POINT('',(12.89,44.116,16.5833640546385));
#53042=CARTESIAN_POINT('Origin',(13.47,44.116,18.29));
#53043=CARTESIAN_POINT('Origin',(13.47,44.696,18.29));
#53044=CARTESIAN_POINT('Origin',(10.42,39.116,15.24));
#53045=CARTESIAN_POINT('',(10.42,39.116,15.24));
#53046=CARTESIAN_POINT('',(16.764,39.116,15.24));
#53047=CARTESIAN_POINT('',(10.42,39.116,15.24));
#53048=CARTESIAN_POINT('',(16.764,39.116,21.34));
#53049=CARTESIAN_POINT('',(16.764,39.116,15.24));
#53050=CARTESIAN_POINT('',(10.42,39.116,21.34));
#53051=CARTESIAN_POINT('',(10.42,39.116,21.34));
#53052=CARTESIAN_POINT('',(10.42,39.116,15.24));
#53053=CARTESIAN_POINT('Origin',(-13.47,44.6575256328986,18.29));
#53054=CARTESIAN_POINT('Ctrl Pts',(-12.89,44.116,19.9966359453615));
#53055=CARTESIAN_POINT('Ctrl Pts',(-13.0870148223526,44.1479198171785,20.0074838910021));
#53056=CARTESIAN_POINT('Ctrl Pts',(-13.282624866759,44.1642087318133,20.012267196773));
#53057=CARTESIAN_POINT('Ctrl Pts',(-13.47,44.1642087318133,20.012267196773));
#53058=CARTESIAN_POINT('Ctrl Pts',(-13.657375133241,44.1642087318133,20.012267196773));
#53059=CARTESIAN_POINT('Ctrl Pts',(-13.8529851776474,44.1479198171785,20.0074838910021));
#53060=CARTESIAN_POINT('Ctrl Pts',(-14.05,44.116,19.9966359453615));
#53061=CARTESIAN_POINT('Origin',(-13.47,44.6575256328986,18.29));
#53062=CARTESIAN_POINT('Ctrl Pts',(-14.05,44.116,16.5833640546385));
#53063=CARTESIAN_POINT('Ctrl Pts',(-13.8529851776474,44.1479198171785,16.5725161089979));
#53064=CARTESIAN_POINT('Ctrl Pts',(-13.657375133241,44.1642087318133,16.567732803227));
#53065=CARTESIAN_POINT('Ctrl Pts',(-13.282624866759,44.1642087318133,16.567732803227));
#53066=CARTESIAN_POINT('Ctrl Pts',(-13.0870148223526,44.1479198171785,16.5725161089979));
#53067=CARTESIAN_POINT('Ctrl Pts',(-12.89,44.116,16.5833640546385));
#53068=CARTESIAN_POINT('Origin',(-16.764,44.696,18.29));
#53069=CARTESIAN_POINT('',(-16.464,44.696,20.0925));
#53070=CARTESIAN_POINT('Origin',(-16.464,44.696,18.29));
#53071=CARTESIAN_POINT('',(-8.964,44.696,20.0925));
#53072=CARTESIAN_POINT('',(-16.764,44.696,20.0925));
#53073=CARTESIAN_POINT('',(-8.964,42.8935,18.29));
#53074=CARTESIAN_POINT('Origin',(-8.964,44.696,18.29));
#53075=CARTESIAN_POINT('Origin',(-8.964,44.696,18.29));
#53076=CARTESIAN_POINT('Origin',(13.47,44.6575256328986,18.29));
#53077=CARTESIAN_POINT('Ctrl Pts',(12.89,44.116,16.5833640546385));
#53078=CARTESIAN_POINT('Ctrl Pts',(13.0870148223526,44.1479198171785,16.5725161089979));
#53079=CARTESIAN_POINT('Ctrl Pts',(13.282624866759,44.1642087318133,16.567732803227));
#53080=CARTESIAN_POINT('Ctrl Pts',(13.47,44.1642087318133,16.567732803227));
#53081=CARTESIAN_POINT('Ctrl Pts',(13.657375133241,44.1642087318133,16.567732803227));
#53082=CARTESIAN_POINT('Ctrl Pts',(13.8529851776474,44.1479198171785,16.5725161089979));
#53083=CARTESIAN_POINT('Ctrl Pts',(14.05,44.116,16.5833640546385));
#53084=CARTESIAN_POINT('Origin',(13.47,44.6575256328986,18.29));
#53085=CARTESIAN_POINT('Ctrl Pts',(14.05,44.116,19.9966359453615));
#53086=CARTESIAN_POINT('Ctrl Pts',(13.8529851776474,44.1479198171785,20.0074838910021));
#53087=CARTESIAN_POINT('Ctrl Pts',(13.657375133241,44.1642087318133,20.012267196773));
#53088=CARTESIAN_POINT('Ctrl Pts',(13.282624866759,44.1642087318133,20.012267196773));
#53089=CARTESIAN_POINT('Ctrl Pts',(13.0870148223526,44.1479198171785,20.0074838910021));
#53090=CARTESIAN_POINT('Ctrl Pts',(12.89,44.116,19.9966359453615));
#53091=CARTESIAN_POINT('Origin',(16.764,44.696,18.29));
#53092=CARTESIAN_POINT('',(16.464,44.696,20.0925));
#53093=CARTESIAN_POINT('Origin',(16.464,44.696,18.29));
#53094=CARTESIAN_POINT('',(8.964,44.696,20.0925));
#53095=CARTESIAN_POINT('',(16.764,44.696,20.0925));
#53096=CARTESIAN_POINT('',(8.964,42.8935,18.29));
#53097=CARTESIAN_POINT('Origin',(8.964,44.696,18.29));
#53098=CARTESIAN_POINT('Origin',(8.964,44.696,18.29));
#53099=CARTESIAN_POINT('Origin',(-16.614,44.696,18.29));
#53100=CARTESIAN_POINT('',(-16.764,44.696,20.3925));
#53101=CARTESIAN_POINT('',(-16.614,44.696,20.2425));
#53102=CARTESIAN_POINT('Origin',(-16.764,44.696,18.29));
#53103=CARTESIAN_POINT('Origin',(-16.764,47.746,15.24));
#53104=CARTESIAN_POINT('',(-16.764,47.746,21.04));
#53105=CARTESIAN_POINT('',(-16.764,47.446,21.34));
#53106=CARTESIAN_POINT('',(-16.764,49.121,19.665));
#53107=CARTESIAN_POINT('',(-16.764,47.746,15.54));
#53108=CARTESIAN_POINT('',(-16.764,47.746,15.24));
#53109=CARTESIAN_POINT('',(-16.764,47.446,15.24));
#53110=CARTESIAN_POINT('',(-16.764,47.596,15.39));
#53111=CARTESIAN_POINT('',(-16.764,47.746,15.24));
#53112=CARTESIAN_POINT('',(-16.764,47.746,21.34));
#53113=CARTESIAN_POINT('Origin',(-8.964,44.696,18.29));
#53114=CARTESIAN_POINT('',(-7.88094873420282,44.696,18.29));
#53115=CARTESIAN_POINT('',(-8.964,42.8935,18.29));
#53116=CARTESIAN_POINT('Origin',(16.614,44.696,18.29));
#53117=CARTESIAN_POINT('',(16.764,44.696,20.3925));
#53118=CARTESIAN_POINT('',(16.614,44.696,20.2425));
#53119=CARTESIAN_POINT('Origin',(16.764,44.696,18.29));
#53120=CARTESIAN_POINT('Origin',(16.764,39.116,15.24));
#53121=CARTESIAN_POINT('',(16.764,47.446,21.34));
#53122=CARTESIAN_POINT('',(16.764,47.746,21.04));
#53123=CARTESIAN_POINT('',(16.764,46.9635,21.8225));
#53124=CARTESIAN_POINT('',(16.764,39.116,21.34));
#53125=CARTESIAN_POINT('',(16.764,47.446,15.24));
#53126=CARTESIAN_POINT('',(16.764,39.116,15.24));
#53127=CARTESIAN_POINT('',(16.764,47.746,15.54));
#53128=CARTESIAN_POINT('',(16.764,45.4385,13.2325));
#53129=CARTESIAN_POINT('',(16.764,47.746,15.24));
#53130=CARTESIAN_POINT('Origin',(8.42247436710141,44.696,18.29));
#53131=CARTESIAN_POINT('',(7.88094873420282,44.696,18.29));
#53132=CARTESIAN_POINT('',(8.42247436710141,43.79475,18.29));
#53133=CARTESIAN_POINT('Origin',(8.382,47.596,21.19));
#53134=CARTESIAN_POINT('',(8.382,47.446,21.34));
#53135=CARTESIAN_POINT('',(8.382,47.746,21.04));
#53136=CARTESIAN_POINT('Origin',(16.764,47.746,15.24));
#53137=CARTESIAN_POINT('',(8.382,47.746,15.54));
#53138=CARTESIAN_POINT('Origin',(8.382,47.596,15.39));
#53139=CARTESIAN_POINT('',(8.382,47.446,15.24));
#53140=CARTESIAN_POINT('Origin',(10.42,41.646,15.24));
#53141=CARTESIAN_POINT('',(10.42,41.646,15.24));
#53142=CARTESIAN_POINT('',(10.42,41.646,15.24));
#53143=CARTESIAN_POINT('',(10.42,41.646,21.34));
#53144=CARTESIAN_POINT('',(10.42,41.646,21.34));
#53145=CARTESIAN_POINT('',(10.42,41.646,15.24));
#53146=CARTESIAN_POINT('Origin',(-10.42,41.646,15.24));
#53147=CARTESIAN_POINT('',(-10.42,41.646,15.24));
#53148=CARTESIAN_POINT('',(-10.42,41.646,15.24));
#53149=CARTESIAN_POINT('',(-10.42,41.646,21.34));
#53150=CARTESIAN_POINT('',(-10.42,41.646,21.34));
#53151=CARTESIAN_POINT('',(-10.42,41.646,15.24));
#53152=CARTESIAN_POINT('Origin',(-10.42,39.116,15.24));
#53153=CARTESIAN_POINT('',(-10.42,39.116,15.24));
#53154=CARTESIAN_POINT('',(-10.42,39.116,21.34));
#53155=CARTESIAN_POINT('Origin',(0.,43.431,21.34));
#53156=CARTESIAN_POINT('Origin',(0.,43.431,15.24));
#83197=UNCERTAINTY_MEASURE_WITH_UNIT(LENGTH_MEASURE(0.01),#83220,
'DISTANCE_ACCURACY_VALUE',
'Maximum model space distance between geometric entities at asserted c
onnectivities');
#83203=UNCERTAINTY_MEASURE_WITH_UNIT(LENGTH_MEASURE(0.01),#83220,
'DISTANCE_ACCURACY_VALUE',
'Maximum model space distance between geometric entities at asserted c
onnectivities');
#83213=(
GEOMETRIC_REPRESENTATION_CONTEXT(3)
GLOBAL_UNCERTAINTY_ASSIGNED_CONTEXT((#83197))
GLOBAL_UNIT_ASSIGNED_CONTEXT((#83220,#83222,#83223))
REPRESENTATION_CONTEXT('','3D')
);
#83219=(
GEOMETRIC_REPRESENTATION_CONTEXT(3)
GLOBAL_UNCERTAINTY_ASSIGNED_CONTEXT((#83203))
GLOBAL_UNIT_ASSIGNED_CONTEXT((#83220,#83222,#83223))
REPRESENTATION_CONTEXT('','3D')
);
#83220=(
LENGTH_UNIT()
NAMED_UNIT(*)
SI_UNIT(.MILLI.,.METRE.)
);
#83222=(
NAMED_UNIT(*)
PLANE_ANGLE_UNIT()
SI_UNIT($,.RADIAN.)
);
#83223=(
NAMED_UNIT(*)
SI_UNIT($,.STERADIAN.)
SOLID_ANGLE_UNIT()
);
#83233=SHAPE_DEFINITION_REPRESENTATION(#83248,#83308);
#83248=PRODUCT_DEFINITION_SHAPE('',$,#83324);
#83308=SHAPE_REPRESENTATION('',(#28406),#83213);
#83314=PRODUCT_DEFINITION_CONTEXT('part definition',#83361,'design');
#83324=PRODUCT_DEFINITION('90 Degree Dual Side Mount',
'90 Degree Dual Side Mount',#83339,#83314);
#83339=PRODUCT_DEFINITION_FORMATION('',$,#83372);
#83361=APPLICATION_CONTEXT(
'Core Data for Automotive Mechanical Design Process');
#83362=PRODUCT_CONTEXT('part definition',#83361,'mechanical');
#83372=PRODUCT('90 Degree Dual Side Mount','90 Degree Dual Side Mount',
$,(#83362));
#83387=PRESENTATION_STYLE_ASSIGNMENT((#83402));
#83402=SURFACE_STYLE_USAGE(.BOTH.,#83417);
#83417=SURFACE_SIDE_STYLE('',(#83432));
#83432=SURFACE_STYLE_FILL_AREA(#83447);
#83447=FILL_AREA_STYLE('Opaque(212,215,220)',(#83462));
#83462=FILL_AREA_STYLE_COLOUR('Opaque(212,215,220)',#83477);
#83477=COLOUR_RGB('Opaque(212,215,220)', 0.40784314, 0.44705882, 0.49803922);
ENDSEC;
END-ISO-10303-21;
